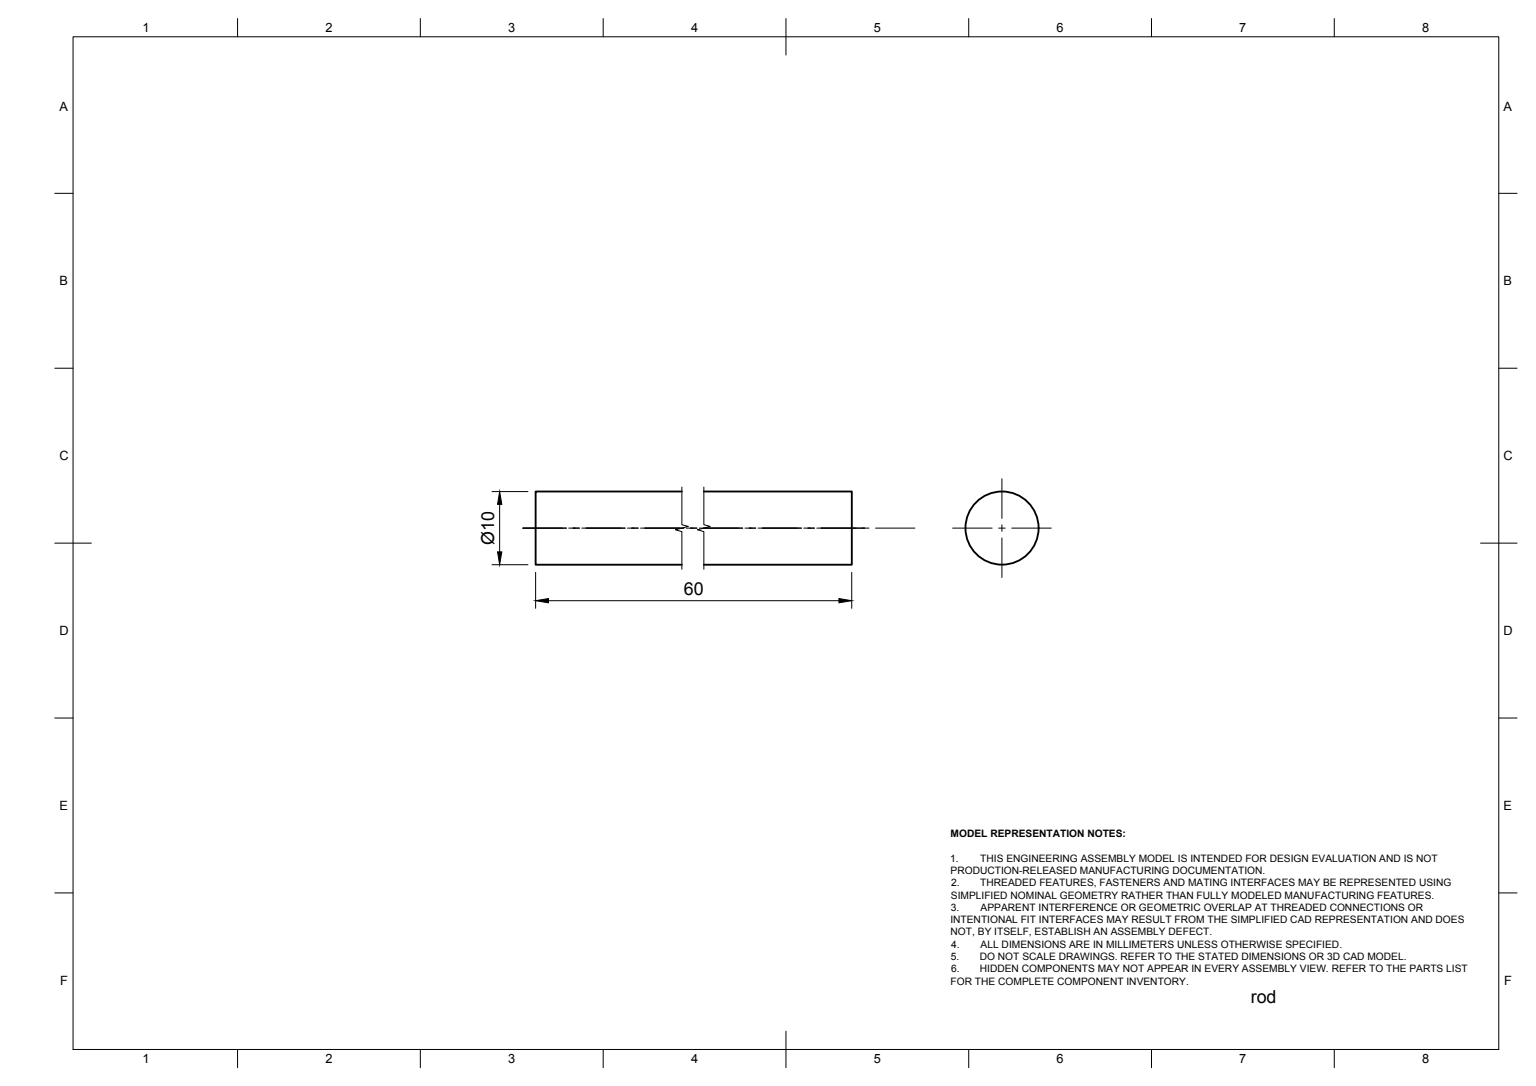
ISO-10303-21;
HEADER;
/* Generated by software containing ST-Developer
 * from STEP Tools, Inc. (www.steptools.com) 
 */

FILE_DESCRIPTION(
/* description */ (''),
/* implementation_level */ '2;1');

FILE_NAME(
/* name */ 'rod.step',
/* time_stamp */ '2026-10-07T11:02:43-07:00',
/* author */ (''),
/* organization */ (''),
/* preprocessor_version */ 'ST-DEVELOPER v20.2',
/* originating_system */ 'Autodesk Translation Framework v15.15.0.0',
/* authorisation */ '');

FILE_SCHEMA (('AUTOMOTIVE_DESIGN { 1 0 10303 214 3 1 1 }'));
ENDSEC;

DATA;
#10=MECHANICAL_DESIGN_GEOMETRIC_PRESENTATION_REPRESENTATION('',(#69),#5505);
#55=SHAPE_REPRESENTATION_RELATIONSHIP('SRR','None',#5540,#62);
#62=ADVANCED_BREP_SHAPE_REPRESENTATION('',(#76),#5501);
#69=STYLED_ITEM('',(#5584),#76);
#76=MANIFOLD_SOLID_BREP('Body1',#3296);
#132=CYLINDRICAL_SURFACE('',#3516,5.);
#194=CIRCLE('',#3515,5.);
#195=CIRCLE('',#3517,5.);
#326=FACE_OUTER_BOUND('',#514,.T.);
#327=FACE_OUTER_BOUND('',#515,.T.);
#328=FACE_OUTER_BOUND('',#516,.T.);
#514=EDGE_LOOP('',(#2600));
#515=EDGE_LOOP('',(#2601,#2602,#2603,#2604));
#516=EDGE_LOOP('',(#2605));
#812=LINE('',#5070,#1182);
#1182=VECTOR('',#4136,5.);
#1509=VERTEX_POINT('',#5065);
#1510=VERTEX_POINT('',#5068);
#1895=EDGE_CURVE('',#1509,#1509,#194,.T.);
#1896=EDGE_CURVE('',#1510,#1510,#195,.T.);
#1897=EDGE_CURVE('',#1510,#1509,#812,.T.);
#2600=ORIENTED_EDGE('',*,*,#1895,.T.);
#2601=ORIENTED_EDGE('',*,*,#1896,.F.);
#2602=ORIENTED_EDGE('',*,*,#1897,.T.);
#2603=ORIENTED_EDGE('',*,*,#1895,.F.);
#2604=ORIENTED_EDGE('',*,*,#1897,.F.);
#2605=ORIENTED_EDGE('',*,*,#1896,.T.);
#3072=PLANE('',#3514);
#3073=PLANE('',#3518);
#3217=ADVANCED_FACE('',(#326),#3072,.F.);
#3218=ADVANCED_FACE('',(#327),#132,.T.);
#3219=ADVANCED_FACE('',(#328),#3073,.T.);
#3296=CLOSED_SHELL('',(#3217,#3218,#3219));
#3513=AXIS2_PLACEMENT_3D('',#5063,#4126,#4127);
#3514=AXIS2_PLACEMENT_3D('',#5064,#4128,#4129);
#3515=AXIS2_PLACEMENT_3D('',#5066,#4130,#4131);
#3516=AXIS2_PLACEMENT_3D('',#5067,#4132,#4133);
#3517=AXIS2_PLACEMENT_3D('',#5069,#4134,#4135);
#3518=AXIS2_PLACEMENT_3D('',#5071,#4137,#4138);
#4126=DIRECTION('axis',(0.,0.,1.));
#4127=DIRECTION('refdir',(1.,0.,0.));
#4128=DIRECTION('center_axis',(-1.,6.12618443423765E-16,1.10412253250333E-15));
#4129=DIRECTION('ref_axis',(1.10412253250334E-15,1.59865984135391E-14,1.));
#4130=DIRECTION('center_axis',(1.,-6.12618443423765E-16,-1.10412253250333E-15));
#4131=DIRECTION('ref_axis',(1.10412253250334E-15,1.59865984135391E-14,1.));
#4132=DIRECTION('center_axis',(-1.,0.,0.));
#4133=DIRECTION('ref_axis',(0.,1.59865984135391E-14,1.));
#4134=DIRECTION('center_axis',(-1.,6.12618443423765E-16,1.10412253250333E-15));
#4135=DIRECTION('ref_axis',(1.10412253250334E-15,1.59865984135391E-14,1.));
#4136=DIRECTION('',(1.,0.,0.));
#4137=DIRECTION('center_axis',(-1.,6.12618443423765E-16,1.10412253250333E-15));
#4138=DIRECTION('ref_axis',(1.10412253250334E-15,1.59865984135391E-14,1.));
#5063=CARTESIAN_POINT('',(0.,0.,0.));
#5064=CARTESIAN_POINT('Origin',(-442.474405060128,1574.77423490353,703.141071318876));
#5065=CARTESIAN_POINT('',(-442.474405060128,1574.77423490353,698.141071318876));
#5066=CARTESIAN_POINT('Origin',(-442.474405060128,1574.77423490353,703.141071318876));
#5067=CARTESIAN_POINT('Origin',(-472.474405060128,1574.77423490353,703.141071318876));
#5068=CARTESIAN_POINT('',(-502.474405060128,1574.77423490353,698.141071318876));
#5069=CARTESIAN_POINT('Origin',(-502.474405060128,1574.77423490353,703.141071318876));
#5070=CARTESIAN_POINT('',(-472.474405060128,1574.77423490353,698.141071318876));
#5071=CARTESIAN_POINT('Origin',(-502.474405060128,1574.77423490353,703.141071318876));
#5492=UNCERTAINTY_MEASURE_WITH_UNIT(LENGTH_MEASURE(0.01),#5506,
'DISTANCE_ACCURACY_VALUE',
'Maximum model space distance between geometric entities at asserted c
onnectivities');
#5496=UNCERTAINTY_MEASURE_WITH_UNIT(LENGTH_MEASURE(0.01),#5506,
'DISTANCE_ACCURACY_VALUE',
'Maximum model space distance between geometric entities at asserted c
onnectivities');
#5501=(
GEOMETRIC_REPRESENTATION_CONTEXT(3)
GLOBAL_UNCERTAINTY_ASSIGNED_CONTEXT((#5492))
GLOBAL_UNIT_ASSIGNED_CONTEXT((#5506,#5508,#5509))
REPRESENTATION_CONTEXT('','3D')
);
#5505=(
GEOMETRIC_REPRESENTATION_CONTEXT(3)
GLOBAL_UNCERTAINTY_ASSIGNED_CONTEXT((#5496))
GLOBAL_UNIT_ASSIGNED_CONTEXT((#5506,#5508,#5509))
REPRESENTATION_CONTEXT('','3D')
);
#5506=(
LENGTH_UNIT()
NAMED_UNIT(*)
SI_UNIT(.MILLI.,.METRE.)
);
#5508=(
NAMED_UNIT(*)
PLANE_ANGLE_UNIT()
SI_UNIT($,.RADIAN.)
);
#5509=(
NAMED_UNIT(*)
SI_UNIT($,.STERADIAN.)
SOLID_ANGLE_UNIT()
);
#5514=SHAPE_DEFINITION_REPRESENTATION(#5522,#5540);
#5522=PRODUCT_DEFINITION_SHAPE('',$,#5549);
#5540=SHAPE_REPRESENTATION('',(#3513),#5501);
#5544=PRODUCT_DEFINITION_CONTEXT('part definition',#5570,'design');
#5549=PRODUCT_DEFINITION('2026-10-07-10-38-52-522','rod',#5557,#5544);
#5557=PRODUCT_DEFINITION_FORMATION('',$,#5576);
#5570=APPLICATION_CONTEXT(
'Core Data for Automotive Mechanical Design Process');
#5571=PRODUCT_CONTEXT('part definition',#5570,'mechanical');
#5576=PRODUCT('2026-10-07-10-38-52-522','rod',$,(#5571));
#5584=PRESENTATION_STYLE_ASSIGNMENT((#5592));
#5592=SURFACE_STYLE_USAGE(.BOTH.,#5600);
#5600=SURFACE_SIDE_STYLE('',(#5608));
#5608=SURFACE_STYLE_FILL_AREA(#5616);
#5616=FILL_AREA_STYLE('Opaque(160,160,160)',(#5624));
#5624=FILL_AREA_STYLE_COLOUR('Opaque(160,160,160)',#5632);
#5632=COLOUR_RGB('Opaque(160,160,160)', 0.40784314, 0.44705882, 0.49803922);
ENDSEC;
END-ISO-10303-21;
